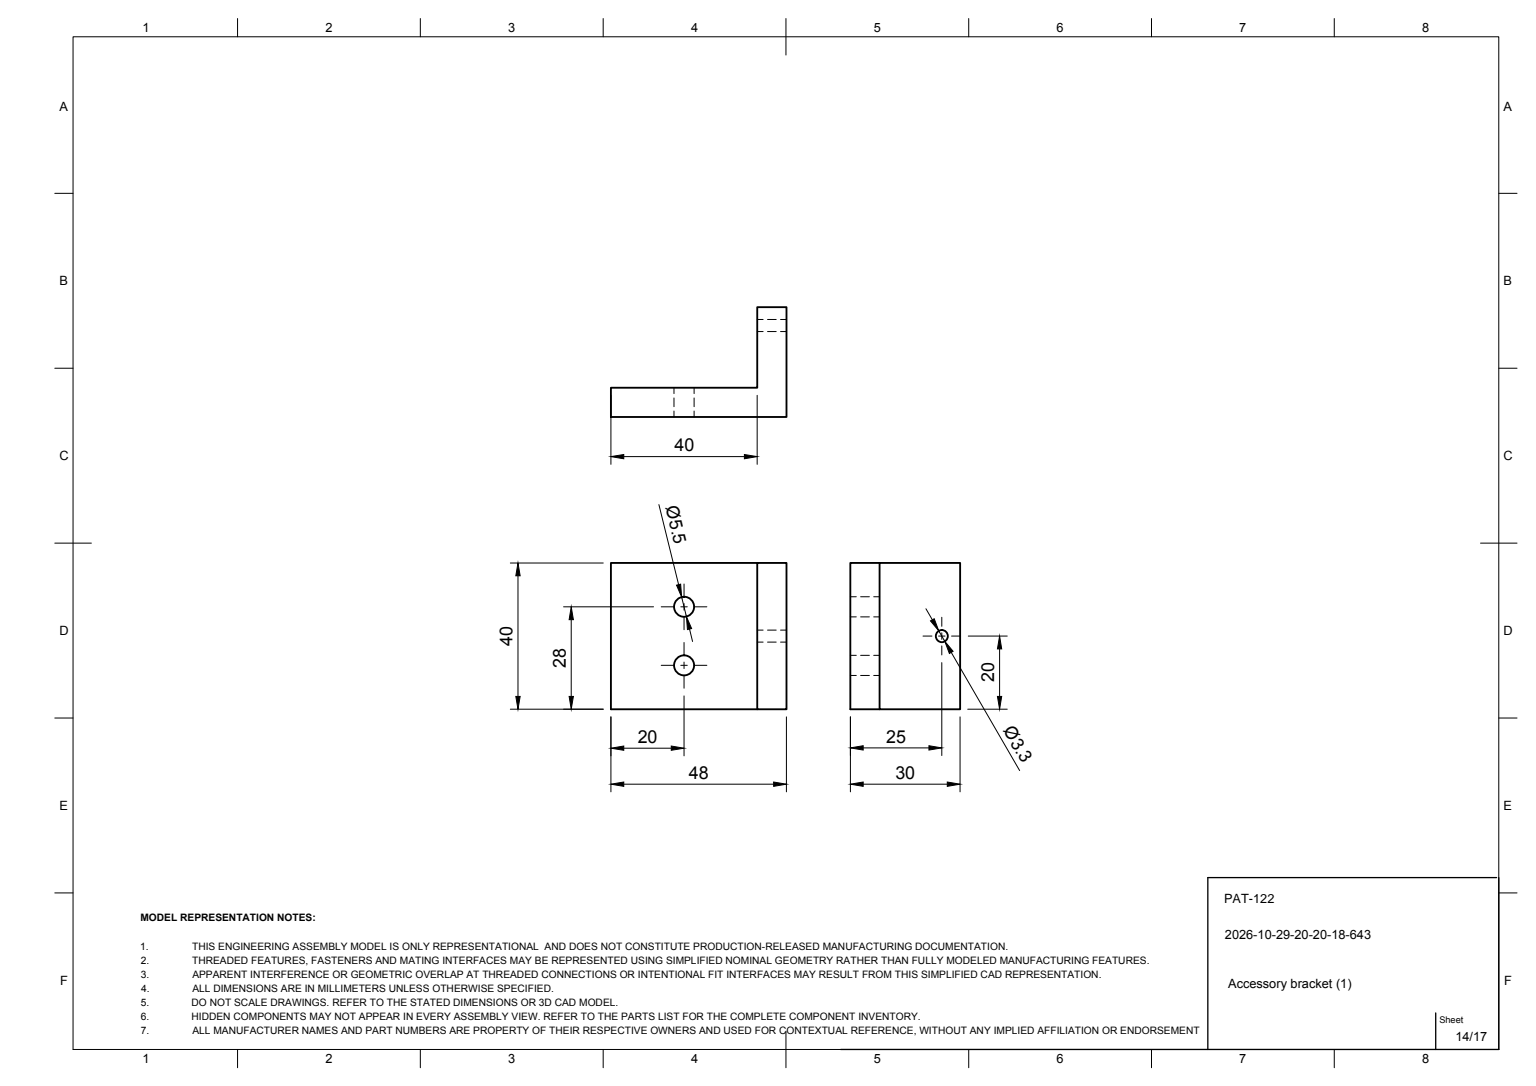
ISO-10303-21;
HEADER;
/* Generated by software containing ST-Developer
 * from STEP Tools, Inc. (www.steptools.com) 
 */

FILE_DESCRIPTION(
/* description */ ('PAT-122'),
/* implementation_level */ '2;1');

FILE_NAME(
/* name */ 'Accessory bracket (1).step',
/* time_stamp */ '2026-10-29T20:20:12-07:00',
/* author */ (''),
/* organization */ (''),
/* preprocessor_version */ 'ST-DEVELOPER v20.2',
/* originating_system */ 'Autodesk Translation Framework v15.17.0.0',
/* authorisation */ '');

FILE_SCHEMA (('AUTOMOTIVE_DESIGN { 1 0 10303 214 3 1 1 }'));
ENDSEC;

DATA;
#10=MECHANICAL_DESIGN_GEOMETRIC_PRESENTATION_REPRESENTATION('',(#502),#10019);
#458=SHAPE_REPRESENTATION_RELATIONSHIP('SRR','None',#10179,#480);
#480=ADVANCED_BREP_SHAPE_REPRESENTATION('',(#524),#10008);
#502=STYLED_ITEM('',(#10327),#524);
#524=MANIFOLD_SOLID_BREP('Body1',#5624);
#573=FACE_BOUND('',#1242,.T.);
#574=FACE_BOUND('',#1245,.T.);
#575=FACE_BOUND('',#1247,.T.);
#576=FACE_BOUND('',#1248,.T.);
#577=FACE_BOUND('',#1251,.T.);
#578=FACE_BOUND('',#1252,.T.);
#657=PLANE('',#6045);
#658=PLANE('',#6046);
#659=PLANE('',#6047);
#660=PLANE('',#6048);
#661=PLANE('',#6049);
#662=PLANE('',#6050);
#663=PLANE('',#6051);
#664=PLANE('',#6052);
#904=FACE_OUTER_BOUND('',#1238,.T.);
#905=FACE_OUTER_BOUND('',#1239,.T.);
#906=FACE_OUTER_BOUND('',#1240,.T.);
#907=FACE_OUTER_BOUND('',#1241,.T.);
#908=FACE_OUTER_BOUND('',#1243,.T.);
#909=FACE_OUTER_BOUND('',#1244,.T.);
#910=FACE_OUTER_BOUND('',#1246,.T.);
#911=FACE_OUTER_BOUND('',#1249,.T.);
#912=FACE_OUTER_BOUND('',#1250,.T.);
#913=FACE_OUTER_BOUND('',#1253,.T.);
#914=FACE_OUTER_BOUND('',#1254,.T.);
#1238=EDGE_LOOP('',(#4183,#4184,#4185,#4186));
#1239=EDGE_LOOP('',(#4187,#4188,#4189,#4190));
#1240=EDGE_LOOP('',(#4191,#4192,#4193,#4194));
#1241=EDGE_LOOP('',(#4195,#4196,#4197,#4198));
#1242=EDGE_LOOP('',(#4199));
#1243=EDGE_LOOP('',(#4200,#4201,#4202,#4203));
#1244=EDGE_LOOP('',(#4204,#4205,#4206,#4207));
#1245=EDGE_LOOP('',(#4208));
#1246=EDGE_LOOP('',(#4209,#4210,#4211,#4212));
#1247=EDGE_LOOP('',(#4213));
#1248=EDGE_LOOP('',(#4214));
#1249=EDGE_LOOP('',(#4215,#4216,#4217,#4218));
#1250=EDGE_LOOP('',(#4219,#4220,#4221,#4222));
#1251=EDGE_LOOP('',(#4223));
#1252=EDGE_LOOP('',(#4224));
#1253=EDGE_LOOP('',(#4225,#4226,#4227,#4228,#4229,#4230));
#1254=EDGE_LOOP('',(#4231,#4232,#4233,#4234,#4235,#4236));
#1584=LINE('',#8419,#2128);
#1585=LINE('',#8425,#2129);
#1586=LINE('',#8431,#2130);
#1587=LINE('',#8436,#2131);
#1588=LINE('',#8438,#2132);
#1589=LINE('',#8440,#2133);
#1590=LINE('',#8441,#2134);
#1591=LINE('',#8444,#2135);
#1592=LINE('',#8446,#2136);
#1593=LINE('',#8447,#2137);
#1594=LINE('',#8450,#2138);
#1595=LINE('',#8452,#2139);
#1596=LINE('',#8453,#2140);
#1597=LINE('',#8456,#2141);
#1598=LINE('',#8458,#2142);
#1599=LINE('',#8459,#2143);
#1600=LINE('',#8462,#2144);
#1601=LINE('',#8464,#2145);
#1602=LINE('',#8465,#2146);
#1603=LINE('',#8467,#2147);
#1604=LINE('',#8468,#2148);
#2128=VECTOR('',#6835,0.164999999999999);
#2129=VECTOR('',#6842,0.275);
#2130=VECTOR('',#6849,0.275);
#2131=VECTOR('',#6854,1.);
#2132=VECTOR('',#6855,1.);
#2133=VECTOR('',#6856,1.);
#2134=VECTOR('',#6857,1.);
#2135=VECTOR('',#6860,1.);
#2136=VECTOR('',#6861,1.);
#2137=VECTOR('',#6862,1.);
#2138=VECTOR('',#6865,1.);
#2139=VECTOR('',#6866,1.);
#2140=VECTOR('',#6867,1.);
#2141=VECTOR('',#6870,1.);
#2142=VECTOR('',#6871,1.);
#2143=VECTOR('',#6872,1.);
#2144=VECTOR('',#6875,1.);
#2145=VECTOR('',#6876,1.);
#2146=VECTOR('',#6877,1.);
#2147=VECTOR('',#6880,1.);
#2148=VECTOR('',#6881,1.);
#2637=CIRCLE('',#6037,0.164999999999999);
#2638=CIRCLE('',#6038,0.164999999999999);
#2639=CIRCLE('',#6040,0.275);
#2640=CIRCLE('',#6041,0.275);
#2641=CIRCLE('',#6043,0.275);
#2642=CIRCLE('',#6044,0.275);
#2811=VERTEX_POINT('',#8416);
#2812=VERTEX_POINT('',#8418);
#2813=VERTEX_POINT('',#8422);
#2814=VERTEX_POINT('',#8424);
#2815=VERTEX_POINT('',#8428);
#2816=VERTEX_POINT('',#8430);
#2817=VERTEX_POINT('',#8434);
#2818=VERTEX_POINT('',#8435);
#2819=VERTEX_POINT('',#8437);
#2820=VERTEX_POINT('',#8439);
#2821=VERTEX_POINT('',#8443);
#2822=VERTEX_POINT('',#8445);
#2823=VERTEX_POINT('',#8449);
#2824=VERTEX_POINT('',#8451);
#2825=VERTEX_POINT('',#8455);
#2826=VERTEX_POINT('',#8457);
#2827=VERTEX_POINT('',#8461);
#2828=VERTEX_POINT('',#8463);
#3326=EDGE_CURVE('',#2811,#2811,#2637,.T.);
#3327=EDGE_CURVE('',#2811,#2812,#1584,.T.);
#3328=EDGE_CURVE('',#2812,#2812,#2638,.T.);
#3329=EDGE_CURVE('',#2813,#2813,#2639,.T.);
#3330=EDGE_CURVE('',#2813,#2814,#1585,.T.);
#3331=EDGE_CURVE('',#2814,#2814,#2640,.T.);
#3332=EDGE_CURVE('',#2815,#2815,#2641,.T.);
#3333=EDGE_CURVE('',#2815,#2816,#1586,.T.);
#3334=EDGE_CURVE('',#2816,#2816,#2642,.T.);
#3335=EDGE_CURVE('',#2817,#2818,#1587,.T.);
#3336=EDGE_CURVE('',#2818,#2819,#1588,.T.);
#3337=EDGE_CURVE('',#2820,#2819,#1589,.T.);
#3338=EDGE_CURVE('',#2817,#2820,#1590,.T.);
#3339=EDGE_CURVE('',#2821,#2817,#1591,.T.);
#3340=EDGE_CURVE('',#2822,#2820,#1592,.T.);
#3341=EDGE_CURVE('',#2821,#2822,#1593,.T.);
#3342=EDGE_CURVE('',#2823,#2821,#1594,.T.);
#3343=EDGE_CURVE('',#2824,#2822,#1595,.T.);
#3344=EDGE_CURVE('',#2823,#2824,#1596,.T.);
#3345=EDGE_CURVE('',#2825,#2823,#1597,.T.);
#3346=EDGE_CURVE('',#2826,#2824,#1598,.T.);
#3347=EDGE_CURVE('',#2825,#2826,#1599,.T.);
#3348=EDGE_CURVE('',#2827,#2825,#1600,.T.);
#3349=EDGE_CURVE('',#2828,#2826,#1601,.T.);
#3350=EDGE_CURVE('',#2827,#2828,#1602,.T.);
#3351=EDGE_CURVE('',#2818,#2827,#1603,.T.);
#3352=EDGE_CURVE('',#2819,#2828,#1604,.T.);
#4183=ORIENTED_EDGE('',*,*,#3326,.F.);
#4184=ORIENTED_EDGE('',*,*,#3327,.T.);
#4185=ORIENTED_EDGE('',*,*,#3328,.F.);
#4186=ORIENTED_EDGE('',*,*,#3327,.F.);
#4187=ORIENTED_EDGE('',*,*,#3329,.F.);
#4188=ORIENTED_EDGE('',*,*,#3330,.T.);
#4189=ORIENTED_EDGE('',*,*,#3331,.F.);
#4190=ORIENTED_EDGE('',*,*,#3330,.F.);
#4191=ORIENTED_EDGE('',*,*,#3332,.F.);
#4192=ORIENTED_EDGE('',*,*,#3333,.T.);
#4193=ORIENTED_EDGE('',*,*,#3334,.F.);
#4194=ORIENTED_EDGE('',*,*,#3333,.F.);
#4195=ORIENTED_EDGE('',*,*,#3335,.T.);
#4196=ORIENTED_EDGE('',*,*,#3336,.T.);
#4197=ORIENTED_EDGE('',*,*,#3337,.F.);
#4198=ORIENTED_EDGE('',*,*,#3338,.F.);
#4199=ORIENTED_EDGE('',*,*,#3328,.T.);
#4200=ORIENTED_EDGE('',*,*,#3339,.T.);
#4201=ORIENTED_EDGE('',*,*,#3338,.T.);
#4202=ORIENTED_EDGE('',*,*,#3340,.F.);
#4203=ORIENTED_EDGE('',*,*,#3341,.F.);
#4204=ORIENTED_EDGE('',*,*,#3342,.T.);
#4205=ORIENTED_EDGE('',*,*,#3341,.T.);
#4206=ORIENTED_EDGE('',*,*,#3343,.F.);
#4207=ORIENTED_EDGE('',*,*,#3344,.F.);
#4208=ORIENTED_EDGE('',*,*,#3326,.T.);
#4209=ORIENTED_EDGE('',*,*,#3345,.T.);
#4210=ORIENTED_EDGE('',*,*,#3344,.T.);
#4211=ORIENTED_EDGE('',*,*,#3346,.F.);
#4212=ORIENTED_EDGE('',*,*,#3347,.F.);
#4213=ORIENTED_EDGE('',*,*,#3331,.T.);
#4214=ORIENTED_EDGE('',*,*,#3334,.T.);
#4215=ORIENTED_EDGE('',*,*,#3348,.T.);
#4216=ORIENTED_EDGE('',*,*,#3347,.T.);
#4217=ORIENTED_EDGE('',*,*,#3349,.F.);
#4218=ORIENTED_EDGE('',*,*,#3350,.F.);
#4219=ORIENTED_EDGE('',*,*,#3351,.T.);
#4220=ORIENTED_EDGE('',*,*,#3350,.T.);
#4221=ORIENTED_EDGE('',*,*,#3352,.F.);
#4222=ORIENTED_EDGE('',*,*,#3336,.F.);
#4223=ORIENTED_EDGE('',*,*,#3329,.T.);
#4224=ORIENTED_EDGE('',*,*,#3332,.T.);
#4225=ORIENTED_EDGE('',*,*,#3352,.T.);
#4226=ORIENTED_EDGE('',*,*,#3349,.T.);
#4227=ORIENTED_EDGE('',*,*,#3346,.T.);
#4228=ORIENTED_EDGE('',*,*,#3343,.T.);
#4229=ORIENTED_EDGE('',*,*,#3340,.T.);
#4230=ORIENTED_EDGE('',*,*,#3337,.T.);
#4231=ORIENTED_EDGE('',*,*,#3351,.F.);
#4232=ORIENTED_EDGE('',*,*,#3335,.F.);
#4233=ORIENTED_EDGE('',*,*,#3339,.F.);
#4234=ORIENTED_EDGE('',*,*,#3342,.F.);
#4235=ORIENTED_EDGE('',*,*,#3345,.F.);
#4236=ORIENTED_EDGE('',*,*,#3348,.F.);
#5292=CYLINDRICAL_SURFACE('',#6036,0.164999999999999);
#5293=CYLINDRICAL_SURFACE('',#6039,0.275);
#5294=CYLINDRICAL_SURFACE('',#6042,0.275);
#5400=ADVANCED_FACE('',(#904),#5292,.F.);
#5401=ADVANCED_FACE('',(#905),#5293,.F.);
#5402=ADVANCED_FACE('',(#906),#5294,.F.);
#5403=ADVANCED_FACE('',(#907,#573),#657,.T.);
#5404=ADVANCED_FACE('',(#908),#658,.T.);
#5405=ADVANCED_FACE('',(#909,#574),#659,.T.);
#5406=ADVANCED_FACE('',(#910,#575,#576),#660,.T.);
#5407=ADVANCED_FACE('',(#911),#661,.T.);
#5408=ADVANCED_FACE('',(#912,#577,#578),#662,.T.);
#5409=ADVANCED_FACE('',(#913),#663,.T.);
#5410=ADVANCED_FACE('',(#914),#664,.F.);
#5624=CLOSED_SHELL('',(#5400,#5401,#5402,#5403,#5404,#5405,#5406,#5407,
#5408,#5409,#5410));
#6035=AXIS2_PLACEMENT_3D('',#8414,#6829,#6830);
#6036=AXIS2_PLACEMENT_3D('',#8415,#6831,#6832);
#6037=AXIS2_PLACEMENT_3D('',#8417,#6833,#6834);
#6038=AXIS2_PLACEMENT_3D('',#8420,#6836,#6837);
#6039=AXIS2_PLACEMENT_3D('',#8421,#6838,#6839);
#6040=AXIS2_PLACEMENT_3D('',#8423,#6840,#6841);
#6041=AXIS2_PLACEMENT_3D('',#8426,#6843,#6844);
#6042=AXIS2_PLACEMENT_3D('',#8427,#6845,#6846);
#6043=AXIS2_PLACEMENT_3D('',#8429,#6847,#6848);
#6044=AXIS2_PLACEMENT_3D('',#8432,#6850,#6851);
#6045=AXIS2_PLACEMENT_3D('',#8433,#6852,#6853);
#6046=AXIS2_PLACEMENT_3D('',#8442,#6858,#6859);
#6047=AXIS2_PLACEMENT_3D('',#8448,#6863,#6864);
#6048=AXIS2_PLACEMENT_3D('',#8454,#6868,#6869);
#6049=AXIS2_PLACEMENT_3D('',#8460,#6873,#6874);
#6050=AXIS2_PLACEMENT_3D('',#8466,#6878,#6879);
#6051=AXIS2_PLACEMENT_3D('',#8469,#6882,#6883);
#6052=AXIS2_PLACEMENT_3D('',#8470,#6884,#6885);
#6829=DIRECTION('axis',(0.,0.,1.));
#6830=DIRECTION('refdir',(1.,0.,0.));
#6831=DIRECTION('center_axis',(0.,0.,1.));
#6832=DIRECTION('ref_axis',(1.,0.,0.));
#6833=DIRECTION('center_axis',(0.,0.,1.));
#6834=DIRECTION('ref_axis',(1.,0.,0.));
#6835=DIRECTION('',(0.,0.,1.));
#6836=DIRECTION('center_axis',(0.,0.,-1.));
#6837=DIRECTION('ref_axis',(1.,0.,0.));
#6838=DIRECTION('center_axis',(0.,1.,0.));
#6839=DIRECTION('ref_axis',(1.,0.,0.));
#6840=DIRECTION('center_axis',(0.,1.,0.));
#6841=DIRECTION('ref_axis',(1.,0.,0.));
#6842=DIRECTION('',(0.,1.,0.));
#6843=DIRECTION('center_axis',(0.,-1.,0.));
#6844=DIRECTION('ref_axis',(1.,0.,0.));
#6845=DIRECTION('center_axis',(0.,1.,0.));
#6846=DIRECTION('ref_axis',(1.,0.,0.));
#6847=DIRECTION('center_axis',(0.,1.,0.));
#6848=DIRECTION('ref_axis',(1.,0.,0.));
#6849=DIRECTION('',(0.,1.,0.));
#6850=DIRECTION('center_axis',(0.,-1.,0.));
#6851=DIRECTION('ref_axis',(1.,0.,0.));
#6852=DIRECTION('center_axis',(0.,0.,1.));
#6853=DIRECTION('ref_axis',(0.,-1.,0.));
#6854=DIRECTION('',(0.,-1.,0.));
#6855=DIRECTION('',(1.,0.,0.));
#6856=DIRECTION('',(0.,-1.,0.));
#6857=DIRECTION('',(1.,0.,0.));
#6858=DIRECTION('center_axis',(0.,1.,0.));
#6859=DIRECTION('ref_axis',(0.,0.,1.));
#6860=DIRECTION('',(0.,0.,1.));
#6861=DIRECTION('',(0.,0.,1.));
#6862=DIRECTION('',(1.,0.,0.));
#6863=DIRECTION('center_axis',(0.,0.,-1.));
#6864=DIRECTION('ref_axis',(0.,1.,0.));
#6865=DIRECTION('',(0.,1.,0.));
#6866=DIRECTION('',(0.,1.,0.));
#6867=DIRECTION('',(1.,0.,0.));
#6868=DIRECTION('center_axis',(0.,1.,0.));
#6869=DIRECTION('ref_axis',(0.,0.,1.));
#6870=DIRECTION('',(0.,0.,1.));
#6871=DIRECTION('',(0.,0.,1.));
#6872=DIRECTION('',(1.,0.,0.));
#6873=DIRECTION('center_axis',(0.,0.,-1.));
#6874=DIRECTION('ref_axis',(0.,1.,0.));
#6875=DIRECTION('',(0.,1.,0.));
#6876=DIRECTION('',(0.,1.,0.));
#6877=DIRECTION('',(1.,0.,0.));
#6878=DIRECTION('center_axis',(0.,-1.,0.));
#6879=DIRECTION('ref_axis',(0.,0.,-1.));
#6880=DIRECTION('',(0.,0.,-1.));
#6881=DIRECTION('',(0.,0.,-1.));
#6882=DIRECTION('center_axis',(1.,0.,0.));
#6883=DIRECTION('ref_axis',(0.,0.,-1.));
#6884=DIRECTION('center_axis',(1.,0.,0.));
#6885=DIRECTION('ref_axis',(0.,0.,-1.));
#8414=CARTESIAN_POINT('',(0.,0.,0.));
#8415=CARTESIAN_POINT('Origin',(10.,22.5,38.9));
#8416=CARTESIAN_POINT('',(9.835,22.5,39.));
#8417=CARTESIAN_POINT('Origin',(10.,22.5,39.));
#8418=CARTESIAN_POINT('',(9.835,22.5,39.8));
#8419=CARTESIAN_POINT('',(9.835,22.5,38.9));
#8420=CARTESIAN_POINT('Origin',(10.,22.5,39.8));
#8421=CARTESIAN_POINT('Origin',(9.2,19.9,37.));
#8422=CARTESIAN_POINT('',(8.925,20.,37.));
#8423=CARTESIAN_POINT('Origin',(9.2,20.,37.));
#8424=CARTESIAN_POINT('',(8.925,20.8,37.));
#8425=CARTESIAN_POINT('',(8.925,19.9,37.));
#8426=CARTESIAN_POINT('Origin',(9.2,20.8,37.));
#8427=CARTESIAN_POINT('Origin',(10.8,19.9,37.));
#8428=CARTESIAN_POINT('',(10.525,20.,37.));
#8429=CARTESIAN_POINT('Origin',(10.8,20.,37.));
#8430=CARTESIAN_POINT('',(10.525,20.8,37.));
#8431=CARTESIAN_POINT('',(10.525,19.9,37.));
#8432=CARTESIAN_POINT('Origin',(10.8,20.8,37.));
#8433=CARTESIAN_POINT('Origin',(8.,23.,39.8));
#8434=CARTESIAN_POINT('',(8.,23.,39.8));
#8435=CARTESIAN_POINT('',(8.,20.,39.8));
#8436=CARTESIAN_POINT('',(8.,23.,39.8));
#8437=CARTESIAN_POINT('',(12.,20.,39.8));
#8438=CARTESIAN_POINT('',(8.,20.,39.8));
#8439=CARTESIAN_POINT('',(12.,23.,39.8));
#8440=CARTESIAN_POINT('',(12.,23.,39.8));
#8441=CARTESIAN_POINT('',(8.,23.,39.8));
#8442=CARTESIAN_POINT('Origin',(8.,23.,39.));
#8443=CARTESIAN_POINT('',(8.,23.,39.));
#8444=CARTESIAN_POINT('',(8.,23.,39.));
#8445=CARTESIAN_POINT('',(12.,23.,39.));
#8446=CARTESIAN_POINT('',(12.,23.,39.));
#8447=CARTESIAN_POINT('',(8.,23.,39.));
#8448=CARTESIAN_POINT('Origin',(8.,20.8,39.));
#8449=CARTESIAN_POINT('',(8.,20.8,39.));
#8450=CARTESIAN_POINT('',(8.,20.8,39.));
#8451=CARTESIAN_POINT('',(12.,20.8,39.));
#8452=CARTESIAN_POINT('',(12.,20.8,39.));
#8453=CARTESIAN_POINT('',(8.,20.8,39.));
#8454=CARTESIAN_POINT('Origin',(8.,20.8,35.));
#8455=CARTESIAN_POINT('',(8.,20.8,35.));
#8456=CARTESIAN_POINT('',(8.,20.8,35.));
#8457=CARTESIAN_POINT('',(12.,20.8,35.));
#8458=CARTESIAN_POINT('',(12.,20.8,35.));
#8459=CARTESIAN_POINT('',(8.,20.8,35.));
#8460=CARTESIAN_POINT('Origin',(8.,20.,35.));
#8461=CARTESIAN_POINT('',(8.,20.,35.));
#8462=CARTESIAN_POINT('',(8.,20.,35.));
#8463=CARTESIAN_POINT('',(12.,20.,35.));
#8464=CARTESIAN_POINT('',(12.,20.,35.));
#8465=CARTESIAN_POINT('',(8.,20.,35.));
#8466=CARTESIAN_POINT('Origin',(8.,20.,39.8));
#8467=CARTESIAN_POINT('',(8.,20.,39.8));
#8468=CARTESIAN_POINT('',(12.,20.,39.8));
#8469=CARTESIAN_POINT('Origin',(12.,21.5,37.4));
#8470=CARTESIAN_POINT('Origin',(8.,21.5,37.4));
#9984=UNCERTAINTY_MEASURE_WITH_UNIT(LENGTH_MEASURE(0.001),#10020,
'DISTANCE_ACCURACY_VALUE',
'Maximum model space distance between geometric entities at asserted c
onnectivities');
#9995=UNCERTAINTY_MEASURE_WITH_UNIT(LENGTH_MEASURE(0.001),#10020,
'DISTANCE_ACCURACY_VALUE',
'Maximum model space distance between geometric entities at asserted c
onnectivities');
#10008=(
GEOMETRIC_REPRESENTATION_CONTEXT(3)
GLOBAL_UNCERTAINTY_ASSIGNED_CONTEXT((#9984))
GLOBAL_UNIT_ASSIGNED_CONTEXT((#10020,#10022,#10023))
REPRESENTATION_CONTEXT('','3D')
);
#10019=(
GEOMETRIC_REPRESENTATION_CONTEXT(3)
GLOBAL_UNCERTAINTY_ASSIGNED_CONTEXT((#9995))
GLOBAL_UNIT_ASSIGNED_CONTEXT((#10020,#10022,#10023))
REPRESENTATION_CONTEXT('','3D')
);
#10020=(
LENGTH_UNIT()
NAMED_UNIT(*)
SI_UNIT(.CENTI.,.METRE.)
);
#10022=(
NAMED_UNIT(*)
PLANE_ANGLE_UNIT()
SI_UNIT($,.RADIAN.)
);
#10023=(
NAMED_UNIT(*)
SI_UNIT($,.STERADIAN.)
SOLID_ANGLE_UNIT()
);
#10036=SHAPE_DEFINITION_REPRESENTATION(#10059,#10179);
#10059=PRODUCT_DEFINITION_SHAPE('',$,#10203);
#10179=SHAPE_REPRESENTATION('',(#6035),#10008);
#10190=PRODUCT_DEFINITION_CONTEXT('part definition',#10261,'design');
#10203=PRODUCT_DEFINITION('Accessory bracket (1)',
'Accessory bracket (1)',#10226,#10190);
#10226=PRODUCT_DEFINITION_FORMATION('',$,#10275);
#10261=APPLICATION_CONTEXT(
'Core Data for Automotive Mechanical Design Process');
#10262=PRODUCT_CONTEXT('part definition',#10261,'mechanical');
#10275=PRODUCT('Accessory bracket (1)','Accessory bracket (1)',
'Accessory bracket (1)',(#10262));
#10321=COLOUR_RGB('Dark Blue',0.08,0.2,0.34);
#10322=FILL_AREA_STYLE_COLOUR('',#10321);
#10323=FILL_AREA_STYLE('',(#10322));
#10324=SURFACE_STYLE_FILL_AREA(#10323);
#10325=SURFACE_SIDE_STYLE('',(#10324));
#10326=SURFACE_STYLE_USAGE(.BOTH.,#10325);
#10327=PRESENTATION_STYLE_ASSIGNMENT((#10326));
ENDSEC;
END-ISO-10303-21;
